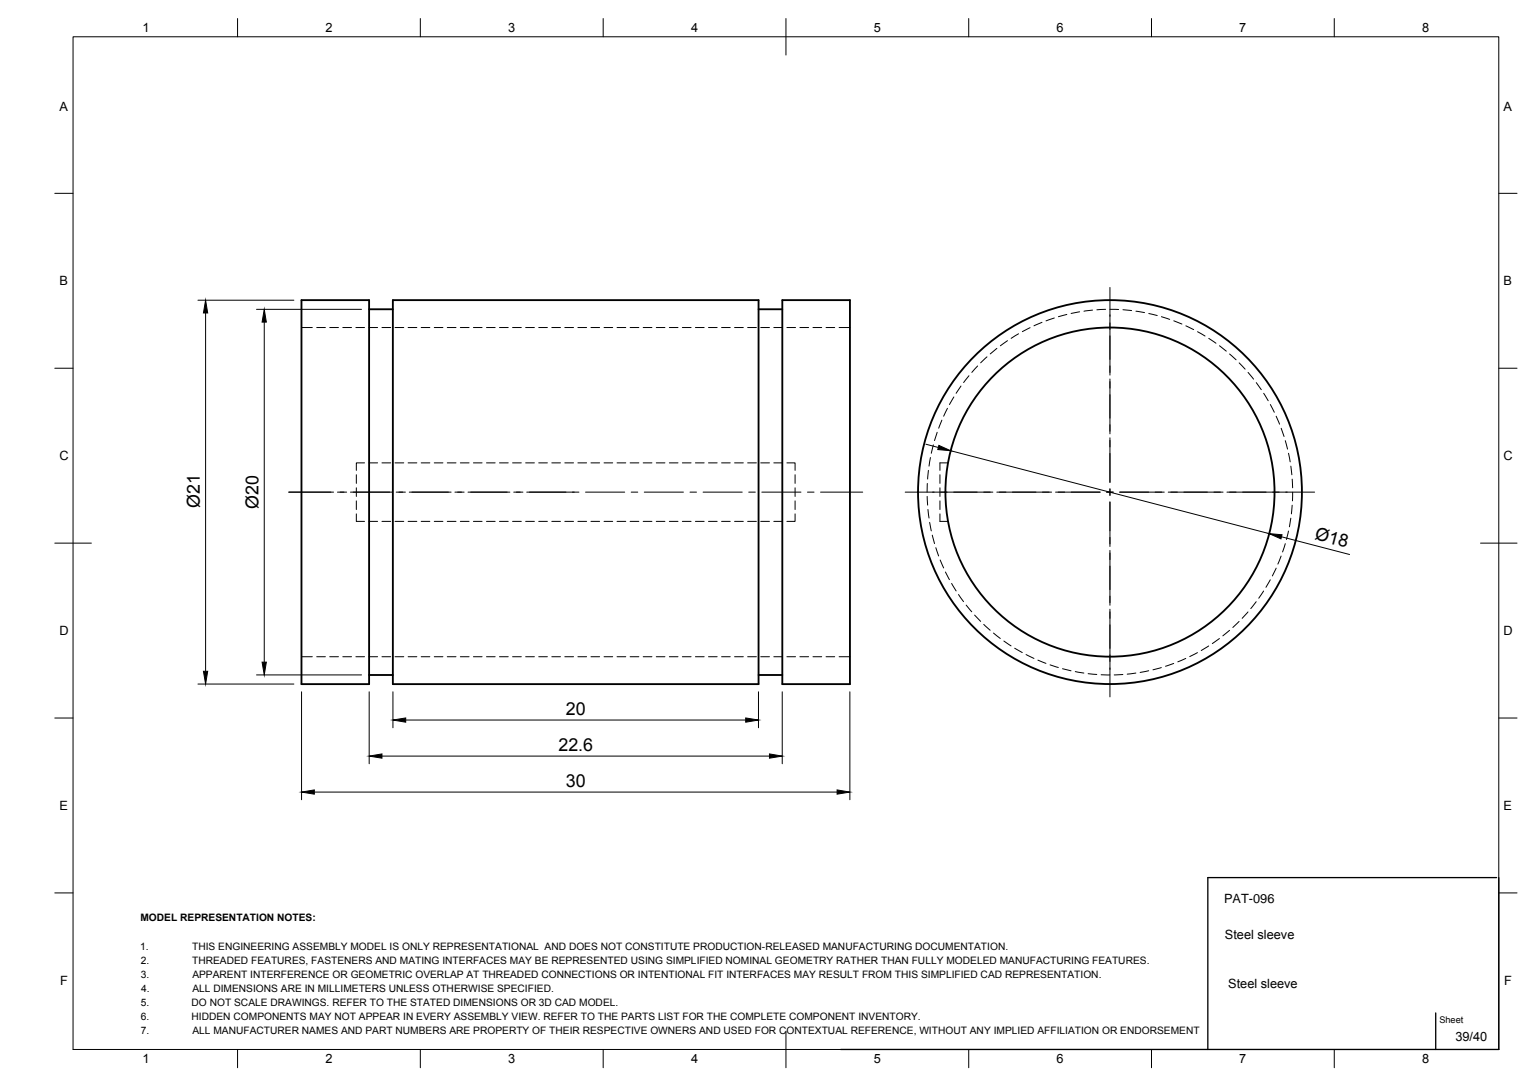
ISO-10303-21;
HEADER;
/* Generated by software containing ST-Developer
 * from STEP Tools, Inc. (www.steptools.com) 
 */

FILE_DESCRIPTION(
/* description */ ('PAT-096'),
/* implementation_level */ '2;1');

FILE_NAME(
/* name */ 'Steel sleeve.step',
/* time_stamp */ '2026-10-29T17:03:14-07:00',
/* author */ (''),
/* organization */ (''),
/* preprocessor_version */ 'ST-DEVELOPER v20.2',
/* originating_system */ 'Autodesk Translation Framework v15.17.0.0',
/* authorisation */ '');

FILE_SCHEMA (('AUTOMOTIVE_DESIGN { 1 0 10303 214 3 1 1 }'));
ENDSEC;

DATA;
#10=MECHANICAL_DESIGN_GEOMETRIC_PRESENTATION_REPRESENTATION('',(#431),#10650);
#361=SHAPE_REPRESENTATION_RELATIONSHIP('SRR','None',#10826,#392);
#392=ADVANCED_BREP_SHAPE_REPRESENTATION('',(#468),#10644);
#431=STYLED_ITEM('',(#11078),#468);
#468=MANIFOLD_SOLID_BREP('Body1',#5566);
#586=FACE_BOUND('',#1521,.T.);
#587=FACE_BOUND('',#1524,.T.);
#588=FACE_BOUND('',#1527,.T.);
#589=FACE_BOUND('',#1530,.T.);
#590=FACE_BOUND('',#1533,.T.);
#591=FACE_BOUND('',#1536,.T.);
#592=FACE_BOUND('',#1538,.T.);
#752=PLANE('',#6504);
#753=PLANE('',#6506);
#754=PLANE('',#6507);
#755=PLANE('',#6509);
#756=PLANE('',#6510);
#757=PLANE('',#6511);
#758=PLANE('',#6516);
#759=PLANE('',#6520);
#760=PLANE('',#6524);
#761=PLANE('',#6528);
#762=PLANE('',#6532);
#1066=FACE_OUTER_BOUND('',#1515,.T.);
#1067=FACE_OUTER_BOUND('',#1516,.T.);
#1068=FACE_OUTER_BOUND('',#1517,.T.);
#1069=FACE_OUTER_BOUND('',#1518,.T.);
#1070=FACE_OUTER_BOUND('',#1519,.T.);
#1071=FACE_OUTER_BOUND('',#1520,.T.);
#1072=FACE_OUTER_BOUND('',#1522,.T.);
#1073=FACE_OUTER_BOUND('',#1523,.T.);
#1074=FACE_OUTER_BOUND('',#1525,.T.);
#1075=FACE_OUTER_BOUND('',#1526,.T.);
#1076=FACE_OUTER_BOUND('',#1528,.T.);
#1077=FACE_OUTER_BOUND('',#1529,.T.);
#1078=FACE_OUTER_BOUND('',#1531,.T.);
#1079=FACE_OUTER_BOUND('',#1532,.T.);
#1080=FACE_OUTER_BOUND('',#1534,.T.);
#1081=FACE_OUTER_BOUND('',#1535,.T.);
#1082=FACE_OUTER_BOUND('',#1537,.T.);
#1515=EDGE_LOOP('',(#4839,#4840,#4841,#4842));
#1516=EDGE_LOOP('',(#4843,#4844,#4845,#4846));
#1517=EDGE_LOOP('',(#4847,#4848,#4849,#4850));
#1518=EDGE_LOOP('',(#4851,#4852,#4853,#4854));
#1519=EDGE_LOOP('',(#4855,#4856,#4857,#4858));
#1520=EDGE_LOOP('',(#4859));
#1521=EDGE_LOOP('',(#4860));
#1522=EDGE_LOOP('',(#4861,#4862,#4863,#4864));
#1523=EDGE_LOOP('',(#4865));
#1524=EDGE_LOOP('',(#4866));
#1525=EDGE_LOOP('',(#4867,#4868,#4869,#4870));
#1526=EDGE_LOOP('',(#4871));
#1527=EDGE_LOOP('',(#4872));
#1528=EDGE_LOOP('',(#4873,#4874,#4875,#4876));
#1529=EDGE_LOOP('',(#4877));
#1530=EDGE_LOOP('',(#4878));
#1531=EDGE_LOOP('',(#4879,#4880,#4881,#4882));
#1532=EDGE_LOOP('',(#4883));
#1533=EDGE_LOOP('',(#4884));
#1534=EDGE_LOOP('',(#4885,#4886,#4887,#4888));
#1535=EDGE_LOOP('',(#4889));
#1536=EDGE_LOOP('',(#4890));
#1537=EDGE_LOOP('',(#4891,#4892,#4893,#4894));
#1538=EDGE_LOOP('',(#4895,#4896,#4897,#4898));
#1860=LINE('',#10264,#2189);
#1861=LINE('',#10266,#2190);
#1862=LINE('',#10267,#2191);
#1863=LINE('',#10270,#2192);
#1864=LINE('',#10272,#2193);
#1865=LINE('',#10273,#2194);
#1866=LINE('',#10278,#2195);
#1867=LINE('',#10279,#2196);
#1868=LINE('',#10281,#2197);
#1869=LINE('',#10282,#2198);
#1870=LINE('',#10292,#2199);
#1871=LINE('',#10299,#2200);
#1872=LINE('',#10306,#2201);
#1873=LINE('',#10313,#2202);
#1874=LINE('',#10320,#2203);
#1875=LINE('',#10325,#2204);
#2189=VECTOR('',#8112,1.);
#2190=VECTOR('',#8113,1.);
#2191=VECTOR('',#8114,1.);
#2192=VECTOR('',#8117,1.);
#2193=VECTOR('',#8118,1.);
#2194=VECTOR('',#8119,1.);
#2195=VECTOR('',#8124,1.);
#2196=VECTOR('',#8125,1.);
#2197=VECTOR('',#8128,1.);
#2198=VECTOR('',#8129,1.);
#2199=VECTOR('',#8142,1.05);
#2200=VECTOR('',#8151,1.);
#2201=VECTOR('',#8160,1.05);
#2202=VECTOR('',#8169,1.);
#2203=VECTOR('',#8178,1.05);
#2204=VECTOR('',#8185,0.9);
#2531=CIRCLE('',#6505,0.9);
#2532=CIRCLE('',#6508,0.9);
#2533=CIRCLE('',#6512,1.05);
#2534=CIRCLE('',#6513,0.9);
#2535=CIRCLE('',#6515,1.05);
#2536=CIRCLE('',#6517,1.);
#2537=CIRCLE('',#6519,1.);
#2538=CIRCLE('',#6521,1.05);
#2539=CIRCLE('',#6523,1.05);
#2540=CIRCLE('',#6525,1.);
#2541=CIRCLE('',#6527,1.);
#2542=CIRCLE('',#6529,1.05);
#2543=CIRCLE('',#6531,1.05);
#2544=CIRCLE('',#6533,0.9);
#2959=VERTEX_POINT('',#10260);
#2960=VERTEX_POINT('',#10261);
#2961=VERTEX_POINT('',#10263);
#2962=VERTEX_POINT('',#10265);
#2963=VERTEX_POINT('',#10269);
#2964=VERTEX_POINT('',#10271);
#2965=VERTEX_POINT('',#10275);
#2966=VERTEX_POINT('',#10277);
#2967=VERTEX_POINT('',#10285);
#2968=VERTEX_POINT('',#10287);
#2969=VERTEX_POINT('',#10290);
#2970=VERTEX_POINT('',#10294);
#2971=VERTEX_POINT('',#10297);
#2972=VERTEX_POINT('',#10301);
#2973=VERTEX_POINT('',#10304);
#2974=VERTEX_POINT('',#10308);
#2975=VERTEX_POINT('',#10311);
#2976=VERTEX_POINT('',#10315);
#2977=VERTEX_POINT('',#10318);
#2978=VERTEX_POINT('',#10322);
#3598=EDGE_CURVE('',#2959,#2960,#2531,.T.);
#3599=EDGE_CURVE('',#2961,#2959,#1860,.T.);
#3600=EDGE_CURVE('',#2962,#2961,#1861,.T.);
#3601=EDGE_CURVE('',#2960,#2962,#1862,.T.);
#3602=EDGE_CURVE('',#2960,#2963,#1863,.T.);
#3603=EDGE_CURVE('',#2964,#2962,#1864,.T.);
#3604=EDGE_CURVE('',#2964,#2963,#1865,.T.);
#3605=EDGE_CURVE('',#2963,#2965,#2532,.T.);
#3606=EDGE_CURVE('',#2966,#2964,#1866,.T.);
#3607=EDGE_CURVE('',#2965,#2966,#1867,.T.);
#3608=EDGE_CURVE('',#2965,#2959,#1868,.T.);
#3609=EDGE_CURVE('',#2966,#2961,#1869,.T.);
#3610=EDGE_CURVE('',#2967,#2967,#2533,.T.);
#3611=EDGE_CURVE('',#2968,#2968,#2534,.T.);
#3612=EDGE_CURVE('',#2969,#2969,#2535,.T.);
#3613=EDGE_CURVE('',#2969,#2967,#1870,.T.);
#3614=EDGE_CURVE('',#2970,#2970,#2536,.T.);
#3615=EDGE_CURVE('',#2971,#2971,#2537,.T.);
#3616=EDGE_CURVE('',#2971,#2970,#1871,.T.);
#3617=EDGE_CURVE('',#2972,#2972,#2538,.T.);
#3618=EDGE_CURVE('',#2973,#2973,#2539,.T.);
#3619=EDGE_CURVE('',#2973,#2972,#1872,.T.);
#3620=EDGE_CURVE('',#2974,#2974,#2540,.T.);
#3621=EDGE_CURVE('',#2975,#2975,#2541,.T.);
#3622=EDGE_CURVE('',#2975,#2974,#1873,.T.);
#3623=EDGE_CURVE('',#2976,#2976,#2542,.T.);
#3624=EDGE_CURVE('',#2977,#2977,#2543,.T.);
#3625=EDGE_CURVE('',#2977,#2976,#1874,.T.);
#3626=EDGE_CURVE('',#2978,#2978,#2544,.T.);
#3627=EDGE_CURVE('',#2978,#2968,#1875,.T.);
#4839=ORIENTED_EDGE('',*,*,#3598,.F.);
#4840=ORIENTED_EDGE('',*,*,#3599,.F.);
#4841=ORIENTED_EDGE('',*,*,#3600,.F.);
#4842=ORIENTED_EDGE('',*,*,#3601,.F.);
#4843=ORIENTED_EDGE('',*,*,#3602,.F.);
#4844=ORIENTED_EDGE('',*,*,#3601,.T.);
#4845=ORIENTED_EDGE('',*,*,#3603,.F.);
#4846=ORIENTED_EDGE('',*,*,#3604,.T.);
#4847=ORIENTED_EDGE('',*,*,#3605,.F.);
#4848=ORIENTED_EDGE('',*,*,#3604,.F.);
#4849=ORIENTED_EDGE('',*,*,#3606,.F.);
#4850=ORIENTED_EDGE('',*,*,#3607,.F.);
#4851=ORIENTED_EDGE('',*,*,#3608,.F.);
#4852=ORIENTED_EDGE('',*,*,#3607,.T.);
#4853=ORIENTED_EDGE('',*,*,#3609,.T.);
#4854=ORIENTED_EDGE('',*,*,#3599,.T.);
#4855=ORIENTED_EDGE('',*,*,#3609,.F.);
#4856=ORIENTED_EDGE('',*,*,#3606,.T.);
#4857=ORIENTED_EDGE('',*,*,#3603,.T.);
#4858=ORIENTED_EDGE('',*,*,#3600,.T.);
#4859=ORIENTED_EDGE('',*,*,#3610,.F.);
#4860=ORIENTED_EDGE('',*,*,#3611,.T.);
#4861=ORIENTED_EDGE('',*,*,#3612,.F.);
#4862=ORIENTED_EDGE('',*,*,#3613,.T.);
#4863=ORIENTED_EDGE('',*,*,#3610,.T.);
#4864=ORIENTED_EDGE('',*,*,#3613,.F.);
#4865=ORIENTED_EDGE('',*,*,#3612,.T.);
#4866=ORIENTED_EDGE('',*,*,#3614,.F.);
#4867=ORIENTED_EDGE('',*,*,#3615,.F.);
#4868=ORIENTED_EDGE('',*,*,#3616,.T.);
#4869=ORIENTED_EDGE('',*,*,#3614,.T.);
#4870=ORIENTED_EDGE('',*,*,#3616,.F.);
#4871=ORIENTED_EDGE('',*,*,#3617,.F.);
#4872=ORIENTED_EDGE('',*,*,#3615,.T.);
#4873=ORIENTED_EDGE('',*,*,#3618,.F.);
#4874=ORIENTED_EDGE('',*,*,#3619,.T.);
#4875=ORIENTED_EDGE('',*,*,#3617,.T.);
#4876=ORIENTED_EDGE('',*,*,#3619,.F.);
#4877=ORIENTED_EDGE('',*,*,#3618,.T.);
#4878=ORIENTED_EDGE('',*,*,#3620,.F.);
#4879=ORIENTED_EDGE('',*,*,#3621,.F.);
#4880=ORIENTED_EDGE('',*,*,#3622,.T.);
#4881=ORIENTED_EDGE('',*,*,#3620,.T.);
#4882=ORIENTED_EDGE('',*,*,#3622,.F.);
#4883=ORIENTED_EDGE('',*,*,#3623,.F.);
#4884=ORIENTED_EDGE('',*,*,#3621,.T.);
#4885=ORIENTED_EDGE('',*,*,#3624,.F.);
#4886=ORIENTED_EDGE('',*,*,#3625,.T.);
#4887=ORIENTED_EDGE('',*,*,#3623,.T.);
#4888=ORIENTED_EDGE('',*,*,#3625,.F.);
#4889=ORIENTED_EDGE('',*,*,#3624,.T.);
#4890=ORIENTED_EDGE('',*,*,#3626,.F.);
#4891=ORIENTED_EDGE('',*,*,#3626,.T.);
#4892=ORIENTED_EDGE('',*,*,#3627,.T.);
#4893=ORIENTED_EDGE('',*,*,#3611,.F.);
#4894=ORIENTED_EDGE('',*,*,#3627,.F.);
#4895=ORIENTED_EDGE('',*,*,#3605,.T.);
#4896=ORIENTED_EDGE('',*,*,#3608,.T.);
#4897=ORIENTED_EDGE('',*,*,#3598,.T.);
#4898=ORIENTED_EDGE('',*,*,#3602,.T.);
#5176=CYLINDRICAL_SURFACE('',#6514,1.05);
#5177=CYLINDRICAL_SURFACE('',#6518,1.);
#5178=CYLINDRICAL_SURFACE('',#6522,1.05);
#5179=CYLINDRICAL_SURFACE('',#6526,1.);
#5180=CYLINDRICAL_SURFACE('',#6530,1.05);
#5181=CYLINDRICAL_SURFACE('',#6534,0.9);
#5471=ADVANCED_FACE('',(#1066),#752,.F.);
#5472=ADVANCED_FACE('',(#1067),#753,.F.);
#5473=ADVANCED_FACE('',(#1068),#754,.F.);
#5474=ADVANCED_FACE('',(#1069),#755,.F.);
#5475=ADVANCED_FACE('',(#1070),#756,.F.);
#5476=ADVANCED_FACE('',(#1071,#586),#757,.T.);
#5477=ADVANCED_FACE('',(#1072),#5176,.T.);
#5478=ADVANCED_FACE('',(#1073,#587),#758,.T.);
#5479=ADVANCED_FACE('',(#1074),#5177,.T.);
#5480=ADVANCED_FACE('',(#1075,#588),#759,.T.);
#5481=ADVANCED_FACE('',(#1076),#5178,.T.);
#5482=ADVANCED_FACE('',(#1077,#589),#760,.T.);
#5483=ADVANCED_FACE('',(#1078),#5179,.T.);
#5484=ADVANCED_FACE('',(#1079,#590),#761,.T.);
#5485=ADVANCED_FACE('',(#1080),#5180,.T.);
#5486=ADVANCED_FACE('',(#1081,#591),#762,.T.);
#5487=ADVANCED_FACE('',(#1082,#592),#5181,.F.);
#5566=CLOSED_SHELL('',(#5471,#5472,#5473,#5474,#5475,#5476,#5477,#5478,
#5479,#5480,#5481,#5482,#5483,#5484,#5485,#5486,#5487));
#6503=AXIS2_PLACEMENT_3D('',#10258,#8106,#8107);
#6504=AXIS2_PLACEMENT_3D('',#10259,#8108,#8109);
#6505=AXIS2_PLACEMENT_3D('',#10262,#8110,#8111);
#6506=AXIS2_PLACEMENT_3D('',#10268,#8115,#8116);
#6507=AXIS2_PLACEMENT_3D('',#10274,#8120,#8121);
#6508=AXIS2_PLACEMENT_3D('',#10276,#8122,#8123);
#6509=AXIS2_PLACEMENT_3D('',#10280,#8126,#8127);
#6510=AXIS2_PLACEMENT_3D('',#10283,#8130,#8131);
#6511=AXIS2_PLACEMENT_3D('',#10284,#8132,#8133);
#6512=AXIS2_PLACEMENT_3D('',#10286,#8134,#8135);
#6513=AXIS2_PLACEMENT_3D('',#10288,#8136,#8137);
#6514=AXIS2_PLACEMENT_3D('',#10289,#8138,#8139);
#6515=AXIS2_PLACEMENT_3D('',#10291,#8140,#8141);
#6516=AXIS2_PLACEMENT_3D('',#10293,#8143,#8144);
#6517=AXIS2_PLACEMENT_3D('',#10295,#8145,#8146);
#6518=AXIS2_PLACEMENT_3D('',#10296,#8147,#8148);
#6519=AXIS2_PLACEMENT_3D('',#10298,#8149,#8150);
#6520=AXIS2_PLACEMENT_3D('',#10300,#8152,#8153);
#6521=AXIS2_PLACEMENT_3D('',#10302,#8154,#8155);
#6522=AXIS2_PLACEMENT_3D('',#10303,#8156,#8157);
#6523=AXIS2_PLACEMENT_3D('',#10305,#8158,#8159);
#6524=AXIS2_PLACEMENT_3D('',#10307,#8161,#8162);
#6525=AXIS2_PLACEMENT_3D('',#10309,#8163,#8164);
#6526=AXIS2_PLACEMENT_3D('',#10310,#8165,#8166);
#6527=AXIS2_PLACEMENT_3D('',#10312,#8167,#8168);
#6528=AXIS2_PLACEMENT_3D('',#10314,#8170,#8171);
#6529=AXIS2_PLACEMENT_3D('',#10316,#8172,#8173);
#6530=AXIS2_PLACEMENT_3D('',#10317,#8174,#8175);
#6531=AXIS2_PLACEMENT_3D('',#10319,#8176,#8177);
#6532=AXIS2_PLACEMENT_3D('',#10321,#8179,#8180);
#6533=AXIS2_PLACEMENT_3D('',#10323,#8181,#8182);
#6534=AXIS2_PLACEMENT_3D('',#10324,#8183,#8184);
#8106=DIRECTION('axis',(0.,0.,1.));
#8107=DIRECTION('refdir',(1.,0.,0.));
#8108=DIRECTION('center_axis',(0.,1.,0.));
#8109=DIRECTION('ref_axis',(0.,0.,1.));
#8110=DIRECTION('center_axis',(0.,-1.,0.));
#8111=DIRECTION('ref_axis',(1.,0.,0.));
#8112=DIRECTION('',(-1.,0.,0.));
#8113=DIRECTION('',(0.,0.,-1.));
#8114=DIRECTION('',(1.,0.,0.));
#8115=DIRECTION('center_axis',(0.,0.,1.));
#8116=DIRECTION('ref_axis',(1.,0.,0.));
#8117=DIRECTION('',(0.,-1.,0.));
#8118=DIRECTION('',(0.,1.,0.));
#8119=DIRECTION('',(-1.,0.,0.));
#8120=DIRECTION('center_axis',(0.,-1.,0.));
#8121=DIRECTION('ref_axis',(0.,0.,-1.));
#8122=DIRECTION('center_axis',(0.,1.,0.));
#8123=DIRECTION('ref_axis',(1.,0.,0.));
#8124=DIRECTION('',(0.,0.,1.));
#8125=DIRECTION('',(1.,0.,0.));
#8126=DIRECTION('center_axis',(0.,0.,-1.));
#8127=DIRECTION('ref_axis',(-1.,0.,0.));
#8128=DIRECTION('',(0.,1.,0.));
#8129=DIRECTION('',(0.,1.,0.));
#8130=DIRECTION('center_axis',(1.,0.,0.));
#8131=DIRECTION('ref_axis',(0.,0.,-1.));
#8132=DIRECTION('center_axis',(0.,1.,0.));
#8133=DIRECTION('ref_axis',(0.,0.,1.));
#8134=DIRECTION('center_axis',(0.,-1.,0.));
#8135=DIRECTION('ref_axis',(1.,0.,0.));
#8136=DIRECTION('center_axis',(0.,-1.,0.));
#8137=DIRECTION('ref_axis',(1.,0.,0.));
#8138=DIRECTION('center_axis',(0.,-1.,0.));
#8139=DIRECTION('ref_axis',(1.,0.,0.));
#8140=DIRECTION('center_axis',(0.,-1.,0.));
#8141=DIRECTION('ref_axis',(1.,0.,0.));
#8142=DIRECTION('',(0.,1.,0.));
#8143=DIRECTION('center_axis',(0.,-1.,0.));
#8144=DIRECTION('ref_axis',(0.,0.,-1.));
#8145=DIRECTION('center_axis',(0.,-1.,0.));
#8146=DIRECTION('ref_axis',(1.,0.,0.));
#8147=DIRECTION('center_axis',(0.,-1.,0.));
#8148=DIRECTION('ref_axis',(1.,0.,0.));
#8149=DIRECTION('center_axis',(0.,-1.,0.));
#8150=DIRECTION('ref_axis',(1.,0.,0.));
#8151=DIRECTION('',(0.,1.,0.));
#8152=DIRECTION('center_axis',(0.,1.,0.));
#8153=DIRECTION('ref_axis',(0.,0.,1.));
#8154=DIRECTION('center_axis',(0.,-1.,0.));
#8155=DIRECTION('ref_axis',(1.,0.,0.));
#8156=DIRECTION('center_axis',(0.,-1.,0.));
#8157=DIRECTION('ref_axis',(1.,0.,0.));
#8158=DIRECTION('center_axis',(0.,-1.,0.));
#8159=DIRECTION('ref_axis',(1.,0.,0.));
#8160=DIRECTION('',(0.,1.,0.));
#8161=DIRECTION('center_axis',(0.,-1.,0.));
#8162=DIRECTION('ref_axis',(0.,0.,-1.));
#8163=DIRECTION('center_axis',(0.,-1.,0.));
#8164=DIRECTION('ref_axis',(1.,0.,0.));
#8165=DIRECTION('center_axis',(0.,-1.,0.));
#8166=DIRECTION('ref_axis',(1.,0.,0.));
#8167=DIRECTION('center_axis',(0.,-1.,0.));
#8168=DIRECTION('ref_axis',(1.,0.,0.));
#8169=DIRECTION('',(0.,1.,0.));
#8170=DIRECTION('center_axis',(0.,1.,0.));
#8171=DIRECTION('ref_axis',(0.,0.,1.));
#8172=DIRECTION('center_axis',(0.,-1.,0.));
#8173=DIRECTION('ref_axis',(1.,0.,0.));
#8174=DIRECTION('center_axis',(0.,-1.,0.));
#8175=DIRECTION('ref_axis',(1.,0.,0.));
#8176=DIRECTION('center_axis',(0.,-1.,0.));
#8177=DIRECTION('ref_axis',(1.,0.,0.));
#8178=DIRECTION('',(0.,1.,0.));
#8179=DIRECTION('center_axis',(0.,-1.,0.));
#8180=DIRECTION('ref_axis',(0.,0.,-1.));
#8181=DIRECTION('center_axis',(0.,-1.,0.));
#8182=DIRECTION('ref_axis',(1.,0.,0.));
#8183=DIRECTION('center_axis',(0.,-1.,0.));
#8184=DIRECTION('ref_axis',(1.,0.,0.));
#8185=DIRECTION('',(0.,1.,0.));
#10258=CARTESIAN_POINT('',(0.,0.,0.));
#10259=CARTESIAN_POINT('Origin',(0.75,1.2,0.));
#10260=CARTESIAN_POINT('',(0.885663593019381,1.2,-0.16));
#10261=CARTESIAN_POINT('',(0.885663593019381,1.2,0.16));
#10262=CARTESIAN_POINT('Origin',(0.,1.2,0.));
#10263=CARTESIAN_POINT('',(0.93,1.2,-0.16));
#10264=CARTESIAN_POINT('',(0.93,1.2,-0.16));
#10265=CARTESIAN_POINT('',(0.93,1.2,0.16));
#10266=CARTESIAN_POINT('',(0.93,1.2,0.16));
#10267=CARTESIAN_POINT('',(0.57,1.2,0.16));
#10268=CARTESIAN_POINT('Origin',(0.57,0.,0.16));
#10269=CARTESIAN_POINT('',(0.885663593019381,-1.2,0.16));
#10270=CARTESIAN_POINT('',(0.885663593019381,0.,0.16));
#10271=CARTESIAN_POINT('',(0.93,-1.2,0.16));
#10272=CARTESIAN_POINT('',(0.93,0.,0.16));
#10273=CARTESIAN_POINT('',(0.57,-1.2,0.16));
#10274=CARTESIAN_POINT('Origin',(0.75,-1.2,0.));
#10275=CARTESIAN_POINT('',(0.885663593019381,-1.2,-0.16));
#10276=CARTESIAN_POINT('Origin',(0.,-1.2,0.));
#10277=CARTESIAN_POINT('',(0.93,-1.2,-0.16));
#10278=CARTESIAN_POINT('',(0.93,-1.2,0.16));
#10279=CARTESIAN_POINT('',(0.93,-1.2,-0.16));
#10280=CARTESIAN_POINT('Origin',(0.93,0.,-0.16));
#10281=CARTESIAN_POINT('',(0.885663593019381,0.,-0.16));
#10282=CARTESIAN_POINT('',(0.93,0.,-0.16));
#10283=CARTESIAN_POINT('Origin',(0.93,0.,0.16));
#10284=CARTESIAN_POINT('Origin',(1.05,1.5,0.));
#10285=CARTESIAN_POINT('',(-1.05,1.5,-1.28587913910472E-16));
#10286=CARTESIAN_POINT('Origin',(0.,1.5,0.));
#10287=CARTESIAN_POINT('',(-0.9,1.5,-1.10218211923262E-16));
#10288=CARTESIAN_POINT('Origin',(0.,1.5,0.));
#10289=CARTESIAN_POINT('Origin',(0.,1.315,0.));
#10290=CARTESIAN_POINT('',(-1.05,1.13,-1.28587913910472E-16));
#10291=CARTESIAN_POINT('Origin',(0.,1.13,0.));
#10292=CARTESIAN_POINT('',(-1.05,1.315,-1.28587913910472E-16));
#10293=CARTESIAN_POINT('Origin',(1.,1.13,0.));
#10294=CARTESIAN_POINT('',(-1.,1.13,-1.22464679914735E-16));
#10295=CARTESIAN_POINT('Origin',(0.,1.13,0.));
#10296=CARTESIAN_POINT('Origin',(0.,1.065,0.));
#10297=CARTESIAN_POINT('',(-1.,1.,-1.22464679914735E-16));
#10298=CARTESIAN_POINT('Origin',(0.,1.,0.));
#10299=CARTESIAN_POINT('',(-1.,1.065,-1.22464679914735E-16));
#10300=CARTESIAN_POINT('Origin',(1.05,1.,0.));
#10301=CARTESIAN_POINT('',(-1.05,1.,-1.28587913910472E-16));
#10302=CARTESIAN_POINT('Origin',(0.,1.,0.));
#10303=CARTESIAN_POINT('Origin',(0.,0.,0.));
#10304=CARTESIAN_POINT('',(-1.05,-1.,-1.28587913910472E-16));
#10305=CARTESIAN_POINT('Origin',(0.,-1.,0.));
#10306=CARTESIAN_POINT('',(-1.05,0.,-1.28587913910472E-16));
#10307=CARTESIAN_POINT('Origin',(1.,-1.,0.));
#10308=CARTESIAN_POINT('',(-1.,-1.,-1.22464679914735E-16));
#10309=CARTESIAN_POINT('Origin',(0.,-1.,0.));
#10310=CARTESIAN_POINT('Origin',(0.,-1.065,0.));
#10311=CARTESIAN_POINT('',(-1.,-1.13,-1.22464679914735E-16));
#10312=CARTESIAN_POINT('Origin',(0.,-1.13,0.));
#10313=CARTESIAN_POINT('',(-1.,-1.065,-1.22464679914735E-16));
#10314=CARTESIAN_POINT('Origin',(1.05,-1.13,0.));
#10315=CARTESIAN_POINT('',(-1.05,-1.13,-1.28587913910472E-16));
#10316=CARTESIAN_POINT('Origin',(0.,-1.13,0.));
#10317=CARTESIAN_POINT('Origin',(0.,-1.315,0.));
#10318=CARTESIAN_POINT('',(-1.05,-1.5,-1.28587913910472E-16));
#10319=CARTESIAN_POINT('Origin',(0.,-1.5,0.));
#10320=CARTESIAN_POINT('',(-1.05,-1.315,-1.28587913910472E-16));
#10321=CARTESIAN_POINT('Origin',(0.9,-1.5,0.));
#10322=CARTESIAN_POINT('',(-0.9,-1.5,-1.10218211923262E-16));
#10323=CARTESIAN_POINT('Origin',(0.,-1.5,0.));
#10324=CARTESIAN_POINT('Origin',(0.,0.,0.));
#10325=CARTESIAN_POINT('',(-0.9,0.,-1.10218211923262E-16));
#10605=UNCERTAINTY_MEASURE_WITH_UNIT(LENGTH_MEASURE(0.001),#10651,
'DISTANCE_ACCURACY_VALUE',
'Maximum model space distance between geometric entities at asserted c
onnectivities');
#10611=UNCERTAINTY_MEASURE_WITH_UNIT(LENGTH_MEASURE(0.001),#10651,
'DISTANCE_ACCURACY_VALUE',
'Maximum model space distance between geometric entities at asserted c
onnectivities');
#10644=(
GEOMETRIC_REPRESENTATION_CONTEXT(3)
GLOBAL_UNCERTAINTY_ASSIGNED_CONTEXT((#10605))
GLOBAL_UNIT_ASSIGNED_CONTEXT((#10651,#10653,#10654))
REPRESENTATION_CONTEXT('','3D')
);
#10650=(
GEOMETRIC_REPRESENTATION_CONTEXT(3)
GLOBAL_UNCERTAINTY_ASSIGNED_CONTEXT((#10611))
GLOBAL_UNIT_ASSIGNED_CONTEXT((#10651,#10653,#10654))
REPRESENTATION_CONTEXT('','3D')
);
#10651=(
LENGTH_UNIT()
NAMED_UNIT(*)
SI_UNIT(.CENTI.,.METRE.)
);
#10653=(
NAMED_UNIT(*)
PLANE_ANGLE_UNIT()
SI_UNIT($,.RADIAN.)
);
#10654=(
NAMED_UNIT(*)
SI_UNIT($,.STERADIAN.)
SOLID_ANGLE_UNIT()
);
#10687=SHAPE_DEFINITION_REPRESENTATION(#10733,#10826);
#10733=PRODUCT_DEFINITION_SHAPE('',$,#10865);
#10826=SHAPE_REPRESENTATION('',(#6503),#10644);
#10832=PRODUCT_DEFINITION_CONTEXT('part definition',#10948,'design');
#10865=PRODUCT_DEFINITION('Steel sleeve','Steel sleeve',#10903,#10832);
#10903=PRODUCT_DEFINITION_FORMATION('',$,#10982);
#10948=APPLICATION_CONTEXT(
'Core Data for Automotive Mechanical Design Process');
#10949=PRODUCT_CONTEXT('part definition',#10948,'mechanical');
#10982=PRODUCT('Steel sleeve','Steel sleeve','Steel sleeve',(#10949));
#11072=COLOUR_RGB('Off White',0.89,0.88,0.83);
#11073=FILL_AREA_STYLE_COLOUR('',#11072);
#11074=FILL_AREA_STYLE('',(#11073));
#11075=SURFACE_STYLE_FILL_AREA(#11074);
#11076=SURFACE_SIDE_STYLE('',(#11075));
#11077=SURFACE_STYLE_USAGE(.BOTH.,#11076);
#11078=PRESENTATION_STYLE_ASSIGNMENT((#11077));
ENDSEC;
END-ISO-10303-21;
